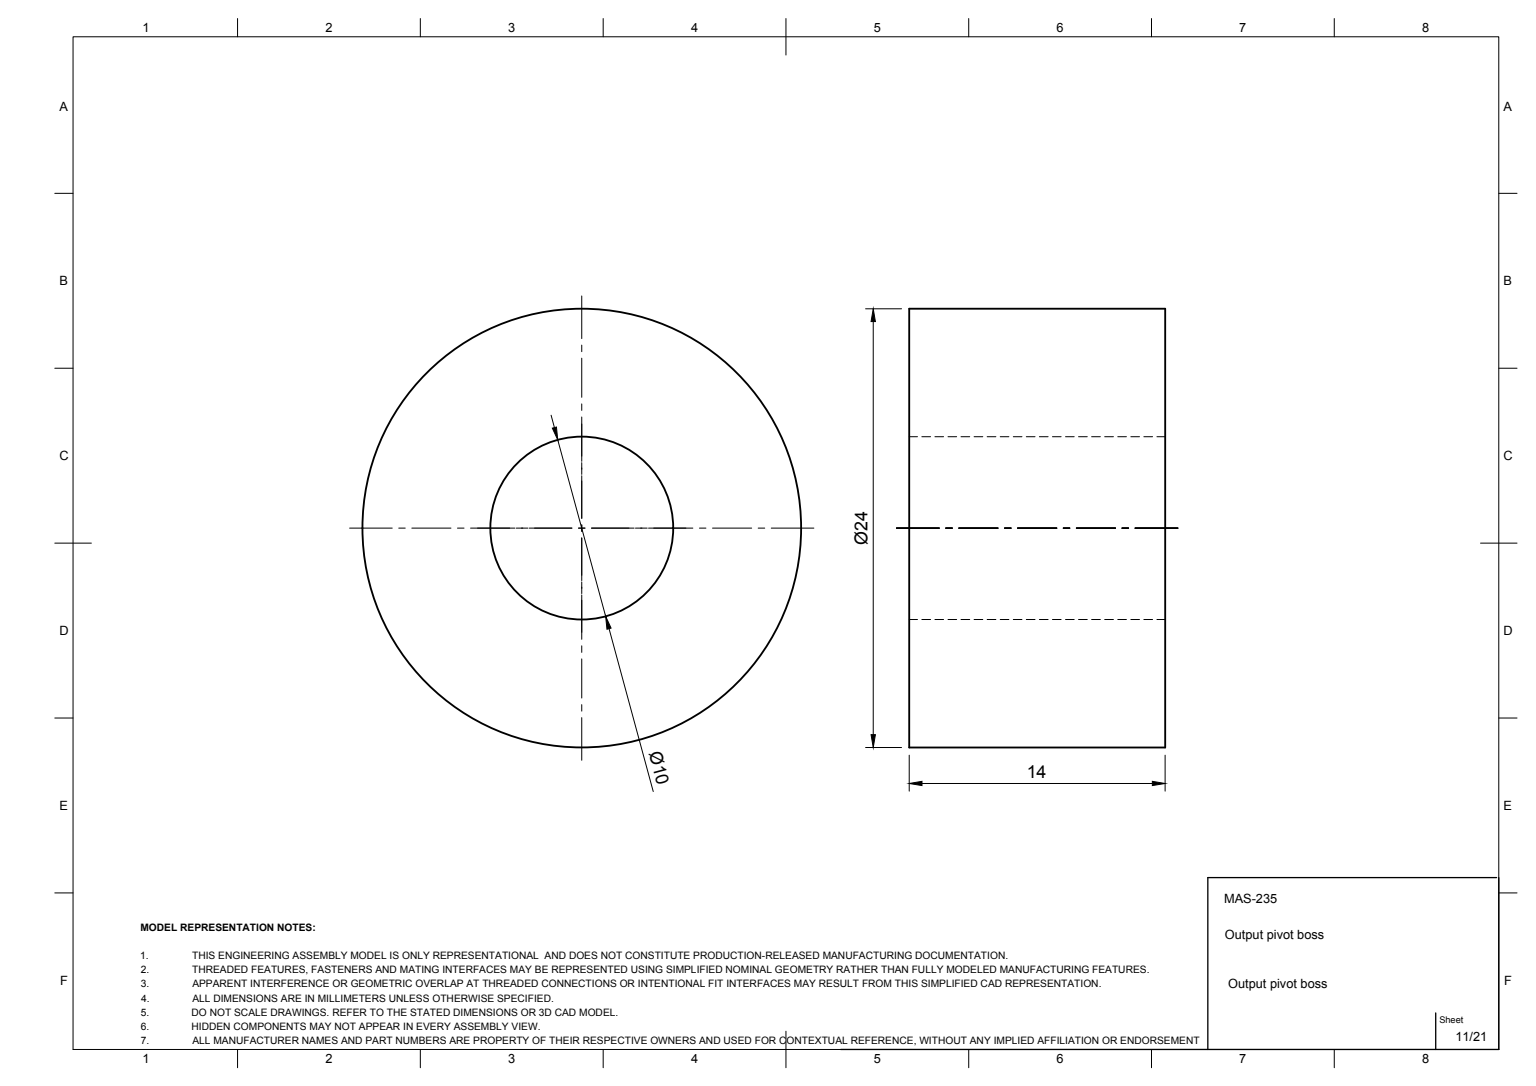
ISO-10303-21;
HEADER;
/* Generated by software containing ST-Developer
 * from STEP Tools, Inc. (www.steptools.com) 
 */

FILE_DESCRIPTION(
/* description */ ('Independent Whitworth quick-return mechanism. Crank radius40, ground-
center spacing80, lever180, connecting rod160, output guide X200. Nomi
nal stroke180 and long/short phase ratio2. Retained guide rods, replac
eable bearing sleeves and captured sliding shoe. No load or production
 rating assigned.'),
/* implementation_level */ '2;1');

FILE_NAME(
/* name */ 'Output pivot boss.step',
/* time_stamp */ '2026-11-09T18:22:56-08:00',
/* author */ (''),
/* organization */ (''),
/* preprocessor_version */ 'ST-DEVELOPER v20.2',
/* originating_system */ 'Autodesk Translation Framework v15.17.0.0',
/* authorisation */ '');

FILE_SCHEMA (('AUTOMOTIVE_DESIGN { 1 0 10303 214 3 1 1 }'));
ENDSEC;

DATA;
#10=MECHANICAL_DESIGN_GEOMETRIC_PRESENTATION_REPRESENTATION('',(#227),#4388);
#187=SHAPE_REPRESENTATION_RELATIONSHIP('SRR','None',#4486,#207);
#207=ADVANCED_BREP_SHAPE_REPRESENTATION('',(#247),#4376);
#227=STYLED_ITEM('',(#4594),#247);
#247=MANIFOLD_SOLID_BREP('Body1',#2332);
#289=FACE_BOUND('',#645,.T.);
#290=FACE_BOUND('',#647,.T.);
#355=PLANE('',#2689);
#356=PLANE('',#2690);
#465=FACE_OUTER_BOUND('',#642,.T.);
#466=FACE_OUTER_BOUND('',#643,.T.);
#467=FACE_OUTER_BOUND('',#644,.T.);
#468=FACE_OUTER_BOUND('',#646,.T.);
#642=EDGE_LOOP('',(#1858,#1859,#1860,#1861));
#643=EDGE_LOOP('',(#1862,#1863,#1864,#1865));
#644=EDGE_LOOP('',(#1866));
#645=EDGE_LOOP('',(#1867));
#646=EDGE_LOOP('',(#1868));
#647=EDGE_LOOP('',(#1869));
#843=LINE('',#3994,#982);
#844=LINE('',#4000,#983);
#982=VECTOR('',#3221,5.);
#983=VECTOR('',#3228,12.);
#1085=CIRCLE('',#2684,5.);
#1086=CIRCLE('',#2685,5.);
#1087=CIRCLE('',#2687,12.);
#1088=CIRCLE('',#2688,12.);
#1247=VERTEX_POINT('',#3991);
#1248=VERTEX_POINT('',#3993);
#1249=VERTEX_POINT('',#3997);
#1250=VERTEX_POINT('',#3999);
#1465=EDGE_CURVE('',#1247,#1247,#1085,.T.);
#1466=EDGE_CURVE('',#1247,#1248,#843,.T.);
#1467=EDGE_CURVE('',#1248,#1248,#1086,.T.);
#1468=EDGE_CURVE('',#1249,#1249,#1087,.T.);
#1469=EDGE_CURVE('',#1249,#1250,#844,.T.);
#1470=EDGE_CURVE('',#1250,#1250,#1088,.T.);
#1858=ORIENTED_EDGE('',*,*,#1465,.F.);
#1859=ORIENTED_EDGE('',*,*,#1466,.T.);
#1860=ORIENTED_EDGE('',*,*,#1467,.T.);
#1861=ORIENTED_EDGE('',*,*,#1466,.F.);
#1862=ORIENTED_EDGE('',*,*,#1468,.F.);
#1863=ORIENTED_EDGE('',*,*,#1469,.T.);
#1864=ORIENTED_EDGE('',*,*,#1470,.T.);
#1865=ORIENTED_EDGE('',*,*,#1469,.F.);
#1866=ORIENTED_EDGE('',*,*,#1468,.T.);
#1867=ORIENTED_EDGE('',*,*,#1465,.T.);
#1868=ORIENTED_EDGE('',*,*,#1470,.F.);
#1869=ORIENTED_EDGE('',*,*,#1467,.F.);
#2140=CYLINDRICAL_SURFACE('',#2683,5.);
#2141=CYLINDRICAL_SURFACE('',#2686,12.);
#2237=ADVANCED_FACE('',(#465),#2140,.F.);
#2238=ADVANCED_FACE('',(#466),#2141,.T.);
#2239=ADVANCED_FACE('',(#467,#289),#355,.T.);
#2240=ADVANCED_FACE('',(#468,#290),#356,.F.);
#2332=CLOSED_SHELL('',(#2237,#2238,#2239,#2240));
#2682=AXIS2_PLACEMENT_3D('',#3989,#3215,#3216);
#2683=AXIS2_PLACEMENT_3D('',#3990,#3217,#3218);
#2684=AXIS2_PLACEMENT_3D('',#3992,#3219,#3220);
#2685=AXIS2_PLACEMENT_3D('',#3995,#3222,#3223);
#2686=AXIS2_PLACEMENT_3D('',#3996,#3224,#3225);
#2687=AXIS2_PLACEMENT_3D('',#3998,#3226,#3227);
#2688=AXIS2_PLACEMENT_3D('',#4001,#3229,#3230);
#2689=AXIS2_PLACEMENT_3D('',#4002,#3231,#3232);
#2690=AXIS2_PLACEMENT_3D('',#4003,#3233,#3234);
#3215=DIRECTION('axis',(0.,0.,1.));
#3216=DIRECTION('refdir',(1.,0.,0.));
#3217=DIRECTION('center_axis',(0.,0.,1.));
#3218=DIRECTION('ref_axis',(1.,0.,0.));
#3219=DIRECTION('center_axis',(0.,0.,-1.));
#3220=DIRECTION('ref_axis',(1.,0.,0.));
#3221=DIRECTION('',(0.,0.,-1.));
#3222=DIRECTION('center_axis',(0.,0.,-1.));
#3223=DIRECTION('ref_axis',(1.,0.,0.));
#3224=DIRECTION('center_axis',(0.,0.,1.));
#3225=DIRECTION('ref_axis',(1.,0.,0.));
#3226=DIRECTION('center_axis',(0.,0.,1.));
#3227=DIRECTION('ref_axis',(1.,0.,0.));
#3228=DIRECTION('',(0.,0.,-1.));
#3229=DIRECTION('center_axis',(0.,0.,1.));
#3230=DIRECTION('ref_axis',(1.,0.,0.));
#3231=DIRECTION('center_axis',(0.,0.,1.));
#3232=DIRECTION('ref_axis',(1.,0.,0.));
#3233=DIRECTION('center_axis',(0.,0.,1.));
#3234=DIRECTION('ref_axis',(1.,0.,0.));
#3989=CARTESIAN_POINT('',(0.,0.,0.));
#3990=CARTESIAN_POINT('Origin',(0.,0.,0.));
#3991=CARTESIAN_POINT('',(-5.,-6.12323399573677E-16,14.));
#3992=CARTESIAN_POINT('Origin',(0.,0.,14.));
#3993=CARTESIAN_POINT('',(-5.,-6.12323399573677E-16,0.));
#3994=CARTESIAN_POINT('',(-5.,-6.12323399573677E-16,0.));
#3995=CARTESIAN_POINT('Origin',(0.,0.,0.));
#3996=CARTESIAN_POINT('Origin',(0.,0.,0.));
#3997=CARTESIAN_POINT('',(-12.,-1.46957615897682E-15,14.));
#3998=CARTESIAN_POINT('Origin',(0.,0.,14.));
#3999=CARTESIAN_POINT('',(-12.,-1.46957615897682E-15,0.));
#4000=CARTESIAN_POINT('',(-12.,-1.46957615897682E-15,0.));
#4001=CARTESIAN_POINT('Origin',(0.,0.,0.));
#4002=CARTESIAN_POINT('Origin',(0.,0.,14.));
#4003=CARTESIAN_POINT('Origin',(0.,0.,0.));
#4354=UNCERTAINTY_MEASURE_WITH_UNIT(LENGTH_MEASURE(0.01),#4389,
'DISTANCE_ACCURACY_VALUE',
'Maximum model space distance between geometric entities at asserted c
onnectivities');
#4366=UNCERTAINTY_MEASURE_WITH_UNIT(LENGTH_MEASURE(0.01),#4389,
'DISTANCE_ACCURACY_VALUE',
'Maximum model space distance between geometric entities at asserted c
onnectivities');
#4376=(
GEOMETRIC_REPRESENTATION_CONTEXT(3)
GLOBAL_UNCERTAINTY_ASSIGNED_CONTEXT((#4354))
GLOBAL_UNIT_ASSIGNED_CONTEXT((#4389,#4391,#4392))
REPRESENTATION_CONTEXT('','3D')
);
#4388=(
GEOMETRIC_REPRESENTATION_CONTEXT(3)
GLOBAL_UNCERTAINTY_ASSIGNED_CONTEXT((#4366))
GLOBAL_UNIT_ASSIGNED_CONTEXT((#4389,#4391,#4392))
REPRESENTATION_CONTEXT('','3D')
);
#4389=(
LENGTH_UNIT()
NAMED_UNIT(*)
SI_UNIT(.MILLI.,.METRE.)
);
#4391=(
NAMED_UNIT(*)
PLANE_ANGLE_UNIT()
SI_UNIT($,.RADIAN.)
);
#4392=(
NAMED_UNIT(*)
SI_UNIT($,.STERADIAN.)
SOLID_ANGLE_UNIT()
);
#4402=SHAPE_DEFINITION_REPRESENTATION(#4423,#4486);
#4423=PRODUCT_DEFINITION_SHAPE('',$,#4508);
#4486=SHAPE_REPRESENTATION('',(#2682),#4376);
#4498=PRODUCT_DEFINITION_CONTEXT('part definition',#4563,'design');
#4508=PRODUCT_DEFINITION('Output pivot boss','Output pivot boss',#4529,
#4498);
#4529=PRODUCT_DEFINITION_FORMATION('',$,#4574);
#4563=APPLICATION_CONTEXT(
'Core Data for Automotive Mechanical Design Process');
#4564=PRODUCT_CONTEXT('part definition',#4563,'mechanical');
#4574=PRODUCT('Output pivot boss','Output pivot boss',$,(#4564));
#4594=PRESENTATION_STYLE_ASSIGNMENT((#4608));
#4608=SURFACE_STYLE_USAGE(.BOTH.,#4622);
#4622=SURFACE_SIDE_STYLE('',(#4636));
#4636=SURFACE_STYLE_FILL_AREA(#4650);
#4650=FILL_AREA_STYLE('Boss gray',(#4664));
#4664=FILL_AREA_STYLE_COLOUR('Boss gray',#4678);
#4678=COLOUR_RGB('Boss gray',0.407843137254902,0.447058823529412,0.498039215686275);
ENDSEC;
END-ISO-10303-21;
